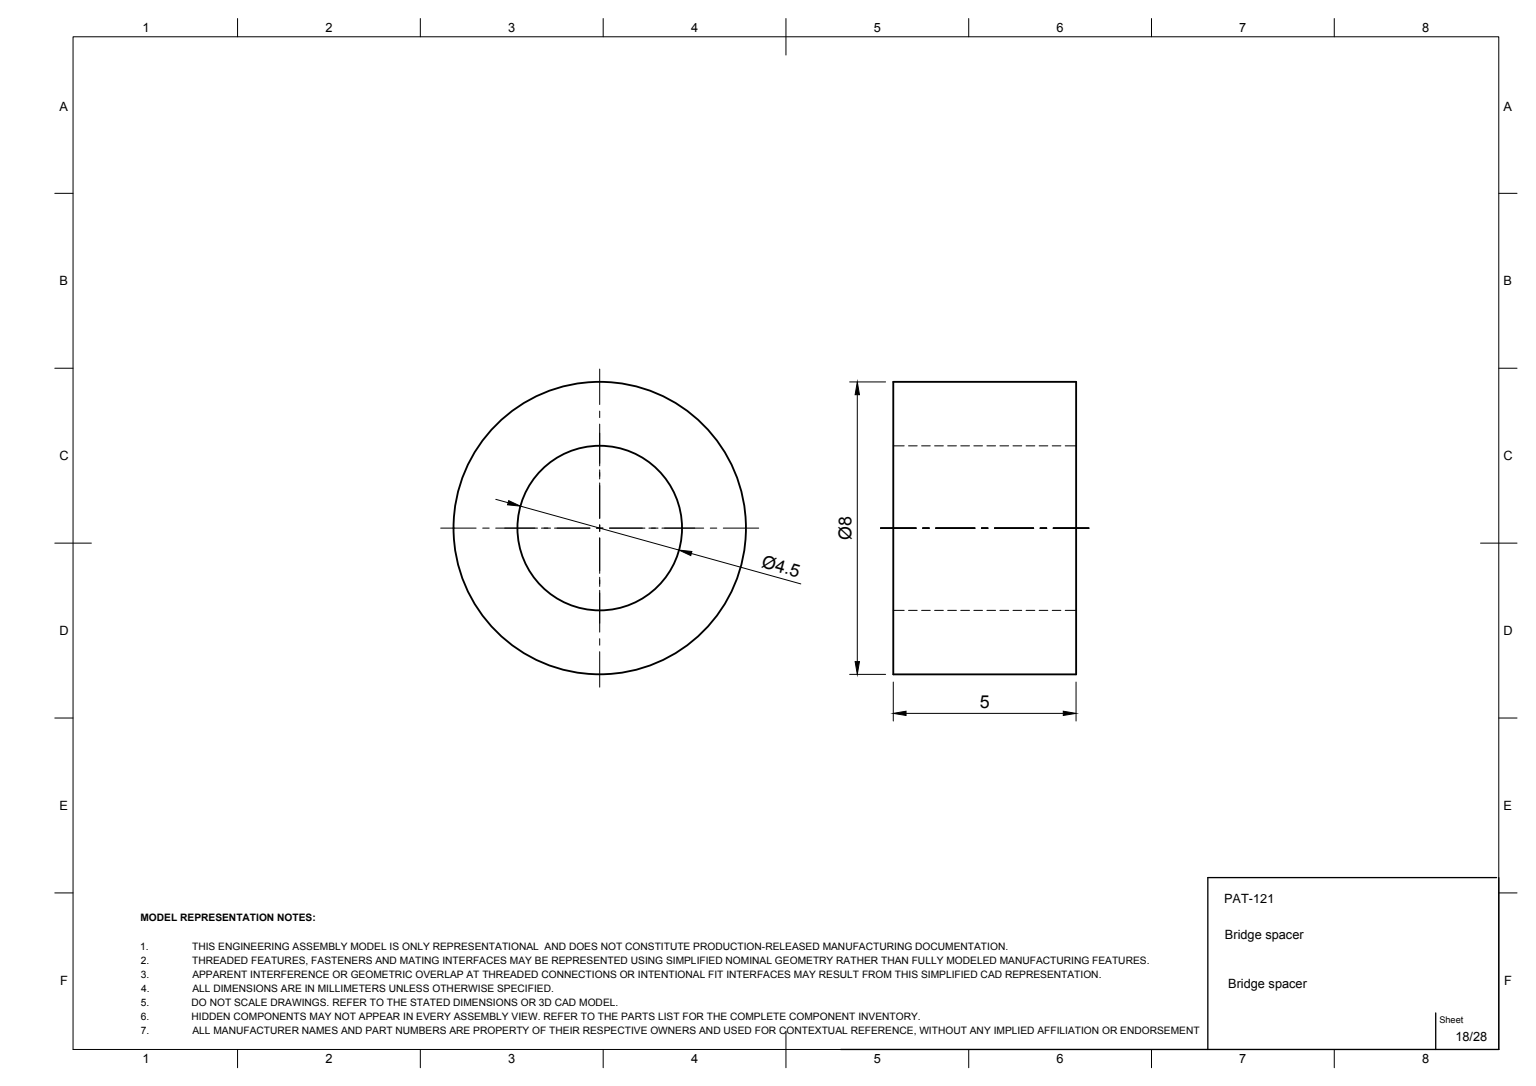
ISO-10303-21;
HEADER;
/* Generated by software containing ST-Developer
 * from STEP Tools, Inc. (www.steptools.com) 
 */

FILE_DESCRIPTION(
/* description */ ('Wall-mounted air drop station'),
/* implementation_level */ '2;1');

FILE_NAME(
/* name */ 'Bridge spacer.step',
/* time_stamp */ '2026-10-28T22:16:19-07:00',
/* author */ (''),
/* organization */ (''),
/* preprocessor_version */ 'ST-DEVELOPER v20.2',
/* originating_system */ 'Autodesk Translation Framework v15.17.0.0',
/* authorisation */ '');

FILE_SCHEMA (('AUTOMOTIVE_DESIGN { 1 0 10303 214 3 1 1 }'));
ENDSEC;

DATA;
#10=MECHANICAL_DESIGN_GEOMETRIC_PRESENTATION_REPRESENTATION('',(#361),#10517);
#303=SHAPE_REPRESENTATION_RELATIONSHIP('SRR','None',#10660,#332);
#332=ADVANCED_BREP_SHAPE_REPRESENTATION('',(#389),#10504);
#361=STYLED_ITEM('',(#10867),#389);
#389=MANIFOLD_SOLID_BREP('Body1',#5901);
#502=FACE_BOUND('',#1439,.T.);
#503=FACE_BOUND('',#1441,.T.);
#661=PLANE('',#6651);
#662=PLANE('',#6652);
#978=FACE_OUTER_BOUND('',#1436,.T.);
#979=FACE_OUTER_BOUND('',#1437,.T.);
#980=FACE_OUTER_BOUND('',#1438,.T.);
#981=FACE_OUTER_BOUND('',#1440,.T.);
#1436=EDGE_LOOP('',(#4905,#4906,#4907,#4908));
#1437=EDGE_LOOP('',(#4909,#4910,#4911,#4912));
#1438=EDGE_LOOP('',(#4913));
#1439=EDGE_LOOP('',(#4914));
#1440=EDGE_LOOP('',(#4915));
#1441=EDGE_LOOP('',(#4916));
#1879=LINE('',#9811,#2343);
#1880=LINE('',#9817,#2344);
#2343=VECTOR('',#8035,0.225);
#2344=VECTOR('',#8042,0.4);
#2687=CIRCLE('',#6646,0.225);
#2688=CIRCLE('',#6647,0.225);
#2689=CIRCLE('',#6649,0.4);
#2690=CIRCLE('',#6650,0.4);
#3073=VERTEX_POINT('',#9808);
#3074=VERTEX_POINT('',#9810);
#3075=VERTEX_POINT('',#9814);
#3076=VERTEX_POINT('',#9816);
#3710=EDGE_CURVE('',#3073,#3073,#2687,.T.);
#3711=EDGE_CURVE('',#3073,#3074,#1879,.T.);
#3712=EDGE_CURVE('',#3074,#3074,#2688,.T.);
#3713=EDGE_CURVE('',#3075,#3075,#2689,.T.);
#3714=EDGE_CURVE('',#3075,#3076,#1880,.T.);
#3715=EDGE_CURVE('',#3076,#3076,#2690,.T.);
#4905=ORIENTED_EDGE('',*,*,#3710,.F.);
#4906=ORIENTED_EDGE('',*,*,#3711,.T.);
#4907=ORIENTED_EDGE('',*,*,#3712,.T.);
#4908=ORIENTED_EDGE('',*,*,#3711,.F.);
#4909=ORIENTED_EDGE('',*,*,#3713,.F.);
#4910=ORIENTED_EDGE('',*,*,#3714,.T.);
#4911=ORIENTED_EDGE('',*,*,#3715,.T.);
#4912=ORIENTED_EDGE('',*,*,#3714,.F.);
#4913=ORIENTED_EDGE('',*,*,#3713,.T.);
#4914=ORIENTED_EDGE('',*,*,#3710,.T.);
#4915=ORIENTED_EDGE('',*,*,#3715,.F.);
#4916=ORIENTED_EDGE('',*,*,#3712,.F.);
#5504=CYLINDRICAL_SURFACE('',#6645,0.225);
#5505=CYLINDRICAL_SURFACE('',#6648,0.4);
#5751=ADVANCED_FACE('',(#978),#5504,.F.);
#5752=ADVANCED_FACE('',(#979),#5505,.T.);
#5753=ADVANCED_FACE('',(#980,#502),#661,.T.);
#5754=ADVANCED_FACE('',(#981,#503),#662,.F.);
#5901=CLOSED_SHELL('',(#5751,#5752,#5753,#5754));
#6644=AXIS2_PLACEMENT_3D('',#9806,#8029,#8030);
#6645=AXIS2_PLACEMENT_3D('',#9807,#8031,#8032);
#6646=AXIS2_PLACEMENT_3D('',#9809,#8033,#8034);
#6647=AXIS2_PLACEMENT_3D('',#9812,#8036,#8037);
#6648=AXIS2_PLACEMENT_3D('',#9813,#8038,#8039);
#6649=AXIS2_PLACEMENT_3D('',#9815,#8040,#8041);
#6650=AXIS2_PLACEMENT_3D('',#9818,#8043,#8044);
#6651=AXIS2_PLACEMENT_3D('',#9819,#8045,#8046);
#6652=AXIS2_PLACEMENT_3D('',#9820,#8047,#8048);
#8029=DIRECTION('axis',(0.,0.,1.));
#8030=DIRECTION('refdir',(1.,0.,0.));
#8031=DIRECTION('center_axis',(0.,0.,1.));
#8032=DIRECTION('ref_axis',(1.,0.,0.));
#8033=DIRECTION('center_axis',(0.,0.,-1.));
#8034=DIRECTION('ref_axis',(1.,0.,0.));
#8035=DIRECTION('',(0.,0.,-1.));
#8036=DIRECTION('center_axis',(0.,0.,-1.));
#8037=DIRECTION('ref_axis',(1.,0.,0.));
#8038=DIRECTION('center_axis',(0.,0.,1.));
#8039=DIRECTION('ref_axis',(1.,0.,0.));
#8040=DIRECTION('center_axis',(0.,0.,1.));
#8041=DIRECTION('ref_axis',(1.,0.,0.));
#8042=DIRECTION('',(0.,0.,-1.));
#8043=DIRECTION('center_axis',(0.,0.,1.));
#8044=DIRECTION('ref_axis',(1.,0.,0.));
#8045=DIRECTION('center_axis',(0.,0.,1.));
#8046=DIRECTION('ref_axis',(1.,0.,0.));
#8047=DIRECTION('center_axis',(0.,0.,1.));
#8048=DIRECTION('ref_axis',(1.,0.,0.));
#9806=CARTESIAN_POINT('',(0.,0.,0.));
#9807=CARTESIAN_POINT('Origin',(-1.3,-1.,7.5));
#9808=CARTESIAN_POINT('',(-1.525,-1.,8.));
#9809=CARTESIAN_POINT('Origin',(-1.3,-1.,8.));
#9810=CARTESIAN_POINT('',(-1.525,-1.,7.5));
#9811=CARTESIAN_POINT('',(-1.525,-1.,7.5));
#9812=CARTESIAN_POINT('Origin',(-1.3,-1.,7.5));
#9813=CARTESIAN_POINT('Origin',(-1.3,-1.,7.5));
#9814=CARTESIAN_POINT('',(-1.7,-1.,8.));
#9815=CARTESIAN_POINT('Origin',(-1.3,-1.,8.));
#9816=CARTESIAN_POINT('',(-1.7,-1.,7.5));
#9817=CARTESIAN_POINT('',(-1.7,-1.,7.5));
#9818=CARTESIAN_POINT('Origin',(-1.3,-1.,7.5));
#9819=CARTESIAN_POINT('Origin',(-1.3,-1.,8.));
#9820=CARTESIAN_POINT('Origin',(-1.3,-1.,7.5));
#10471=UNCERTAINTY_MEASURE_WITH_UNIT(LENGTH_MEASURE(0.001),#10518,
'DISTANCE_ACCURACY_VALUE',
'Maximum model space distance between geometric entities at asserted c
onnectivities');
#10484=UNCERTAINTY_MEASURE_WITH_UNIT(LENGTH_MEASURE(0.001),#10518,
'DISTANCE_ACCURACY_VALUE',
'Maximum model space distance between geometric entities at asserted c
onnectivities');
#10504=(
GEOMETRIC_REPRESENTATION_CONTEXT(3)
GLOBAL_UNCERTAINTY_ASSIGNED_CONTEXT((#10471))
GLOBAL_UNIT_ASSIGNED_CONTEXT((#10518,#10520,#10521))
REPRESENTATION_CONTEXT('','3D')
);
#10517=(
GEOMETRIC_REPRESENTATION_CONTEXT(3)
GLOBAL_UNCERTAINTY_ASSIGNED_CONTEXT((#10484))
GLOBAL_UNIT_ASSIGNED_CONTEXT((#10518,#10520,#10521))
REPRESENTATION_CONTEXT('','3D')
);
#10518=(
LENGTH_UNIT()
NAMED_UNIT(*)
SI_UNIT(.CENTI.,.METRE.)
);
#10520=(
NAMED_UNIT(*)
PLANE_ANGLE_UNIT()
SI_UNIT($,.RADIAN.)
);
#10521=(
NAMED_UNIT(*)
SI_UNIT($,.STERADIAN.)
SOLID_ANGLE_UNIT()
);
#10541=SHAPE_DEFINITION_REPRESENTATION(#10573,#10660);
#10573=PRODUCT_DEFINITION_SHAPE('',$,#10693);
#10660=SHAPE_REPRESENTATION('',(#6644),#10504);
#10673=PRODUCT_DEFINITION_CONTEXT('part definition',#10771,'design');
#10693=PRODUCT_DEFINITION('Bridge spacer','Bridge spacer',#10725,#10673);
#10725=PRODUCT_DEFINITION_FORMATION('',$,#10792);
#10771=APPLICATION_CONTEXT(
'Core Data for Automotive Mechanical Design Process');
#10772=PRODUCT_CONTEXT('part definition',#10771,'mechanical');
#10792=PRODUCT('Bridge spacer','Bridge spacer','Bridge spacer',(#10772));
#10861=COLOUR_RGB('Sky Blue',0.24,0.69,0.87);
#10862=FILL_AREA_STYLE_COLOUR('',#10861);
#10863=FILL_AREA_STYLE('',(#10862));
#10864=SURFACE_STYLE_FILL_AREA(#10863);
#10865=SURFACE_SIDE_STYLE('',(#10864));
#10866=SURFACE_STYLE_USAGE(.BOTH.,#10865);
#10867=PRESENTATION_STYLE_ASSIGNMENT((#10866));
ENDSEC;
END-ISO-10303-21;
